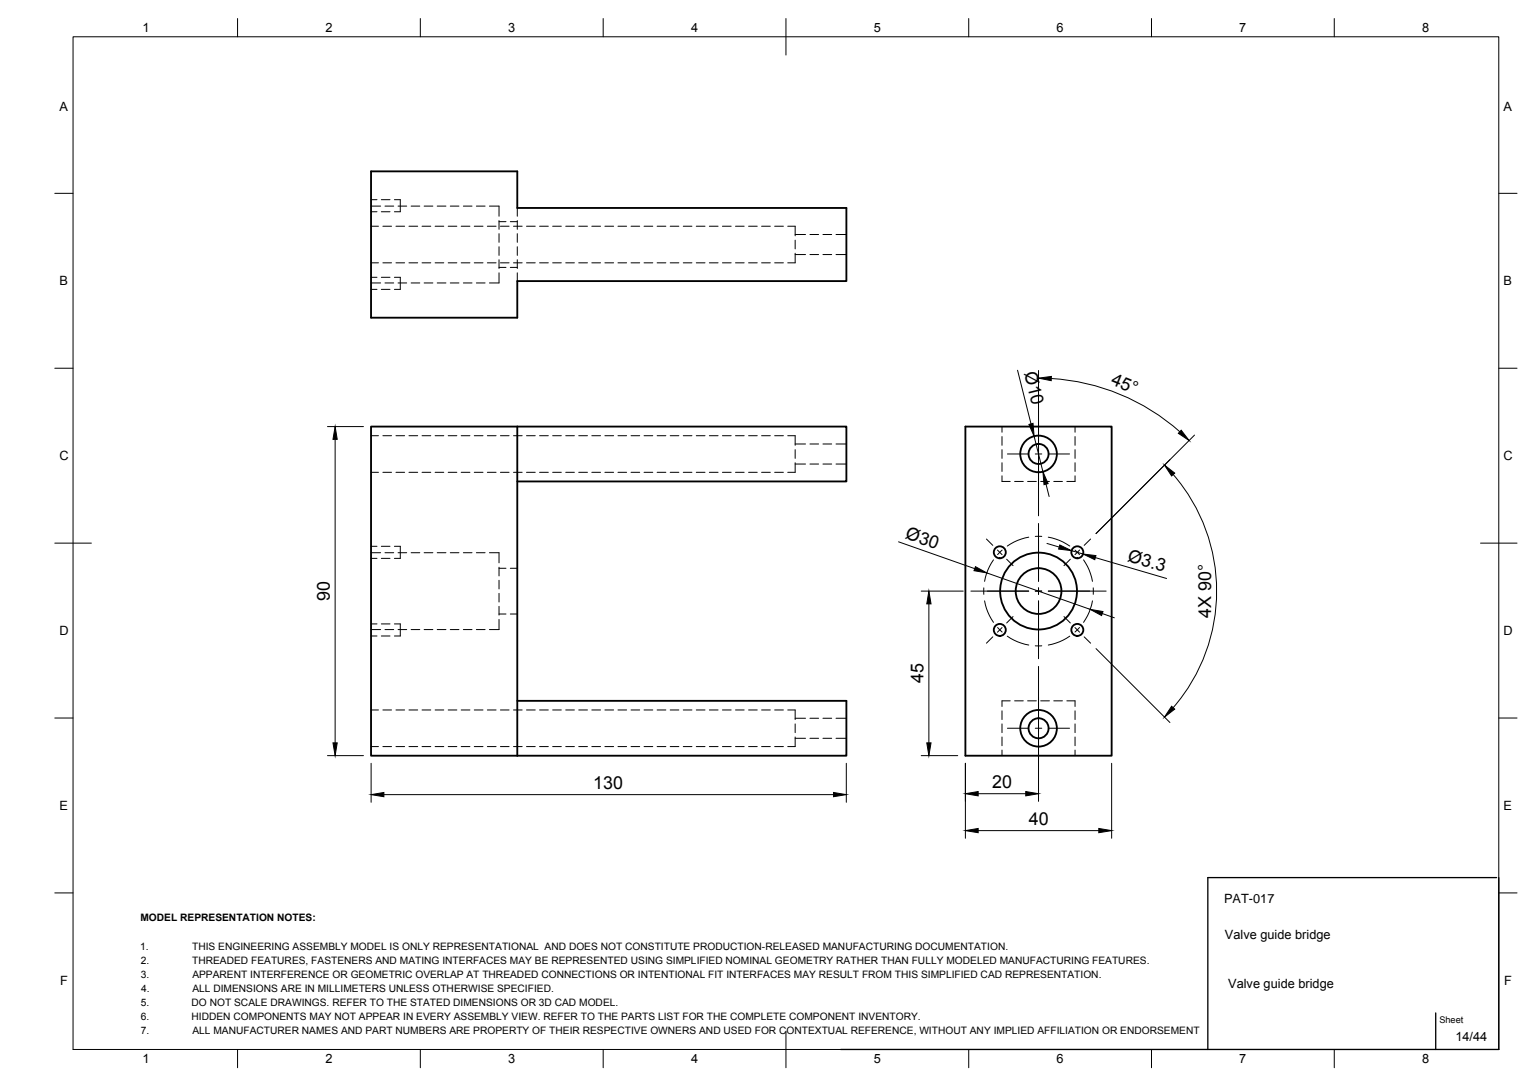
ISO-10303-21;
HEADER;
/* Generated by software containing ST-Developer
 * from STEP Tools, Inc. (www.steptools.com) 
 */

FILE_DESCRIPTION(
/* description */ ('Cam-and-follower valve demonstrator'),
/* implementation_level */ '2;1');

FILE_NAME(
/* name */ 'Valve guide bridge.step',
/* time_stamp */ '2026-10-28T03:25:17-07:00',
/* author */ (''),
/* organization */ (''),
/* preprocessor_version */ 'ST-DEVELOPER v20.2',
/* originating_system */ 'Autodesk Translation Framework v15.17.0.0',
/* authorisation */ '');

FILE_SCHEMA (('AUTOMOTIVE_DESIGN { 1 0 10303 214 3 1 1 }'));
ENDSEC;

DATA;
#10=MECHANICAL_DESIGN_GEOMETRIC_PRESENTATION_REPRESENTATION('',(#421),#12896);
#349=SHAPE_REPRESENTATION_RELATIONSHIP('SRR','None',#13065,#385);
#385=ADVANCED_BREP_SHAPE_REPRESENTATION('',(#464),#12865);
#421=STYLED_ITEM('',(#13323),#464);
#464=MANIFOLD_SOLID_BREP('Body1',#6188);
#580=FACE_BOUND('',#1661,.T.);
#581=FACE_BOUND('',#1665,.T.);
#582=FACE_BOUND('',#1669,.T.);
#583=FACE_BOUND('',#1672,.T.);
#584=FACE_BOUND('',#1678,.T.);
#585=FACE_BOUND('',#1686,.T.);
#586=FACE_BOUND('',#1687,.T.);
#587=FACE_BOUND('',#1688,.T.);
#588=FACE_BOUND('',#1689,.T.);
#589=FACE_BOUND('',#1690,.T.);
#590=FACE_BOUND('',#1691,.T.);
#591=FACE_BOUND('',#1692,.T.);
#592=FACE_BOUND('',#1694,.T.);
#755=CIRCLE('',#6834,0.165);
#756=CIRCLE('',#6835,0.165);
#757=CIRCLE('',#6838,0.165);
#758=CIRCLE('',#6839,0.165);
#759=CIRCLE('',#6842,0.165);
#760=CIRCLE('',#6843,0.165);
#761=CIRCLE('',#6846,0.165);
#762=CIRCLE('',#6847,0.165);
#763=CIRCLE('',#6850,1.05);
#764=CIRCLE('',#6851,1.05);
#765=CIRCLE('',#6853,0.625);
#766=CIRCLE('',#6855,0.625);
#767=CIRCLE('',#6857,0.5);
#768=CIRCLE('',#6858,0.5);
#769=CIRCLE('',#6860,0.275);
#770=CIRCLE('',#6862,0.275);
#771=CIRCLE('',#6864,0.5);
#772=CIRCLE('',#6865,0.5);
#773=CIRCLE('',#6867,0.275);
#774=CIRCLE('',#6869,0.275);
#1021=CYLINDRICAL_SURFACE('',#6833,0.165);
#1022=CYLINDRICAL_SURFACE('',#6837,0.165);
#1023=CYLINDRICAL_SURFACE('',#6841,0.165);
#1024=CYLINDRICAL_SURFACE('',#6845,0.165);
#1025=CYLINDRICAL_SURFACE('',#6849,1.05);
#1026=CYLINDRICAL_SURFACE('',#6854,0.625);
#1027=CYLINDRICAL_SURFACE('',#6856,0.5);
#1028=CYLINDRICAL_SURFACE('',#6861,0.275);
#1029=CYLINDRICAL_SURFACE('',#6863,0.5);
#1030=CYLINDRICAL_SURFACE('',#6868,0.275);
#1198=FACE_OUTER_BOUND('',#1651,.T.);
#1199=FACE_OUTER_BOUND('',#1652,.T.);
#1200=FACE_OUTER_BOUND('',#1653,.T.);
#1201=FACE_OUTER_BOUND('',#1654,.T.);
#1202=FACE_OUTER_BOUND('',#1655,.T.);
#1203=FACE_OUTER_BOUND('',#1656,.T.);
#1204=FACE_OUTER_BOUND('',#1657,.T.);
#1205=FACE_OUTER_BOUND('',#1658,.T.);
#1206=FACE_OUTER_BOUND('',#1659,.T.);
#1207=FACE_OUTER_BOUND('',#1660,.T.);
#1208=FACE_OUTER_BOUND('',#1662,.T.);
#1209=FACE_OUTER_BOUND('',#1663,.T.);
#1210=FACE_OUTER_BOUND('',#1664,.T.);
#1211=FACE_OUTER_BOUND('',#1666,.T.);
#1212=FACE_OUTER_BOUND('',#1667,.T.);
#1213=FACE_OUTER_BOUND('',#1668,.T.);
#1214=FACE_OUTER_BOUND('',#1670,.T.);
#1215=FACE_OUTER_BOUND('',#1671,.T.);
#1216=FACE_OUTER_BOUND('',#1673,.T.);
#1217=FACE_OUTER_BOUND('',#1674,.T.);
#1218=FACE_OUTER_BOUND('',#1675,.T.);
#1219=FACE_OUTER_BOUND('',#1676,.T.);
#1220=FACE_OUTER_BOUND('',#1677,.T.);
#1221=FACE_OUTER_BOUND('',#1679,.T.);
#1222=FACE_OUTER_BOUND('',#1680,.T.);
#1223=FACE_OUTER_BOUND('',#1681,.T.);
#1224=FACE_OUTER_BOUND('',#1682,.T.);
#1225=FACE_OUTER_BOUND('',#1683,.T.);
#1226=FACE_OUTER_BOUND('',#1684,.T.);
#1227=FACE_OUTER_BOUND('',#1685,.T.);
#1228=FACE_OUTER_BOUND('',#1693,.T.);
#1651=EDGE_LOOP('',(#4575,#4576,#4577,#4578));
#1652=EDGE_LOOP('',(#4579));
#1653=EDGE_LOOP('',(#4580,#4581,#4582,#4583));
#1654=EDGE_LOOP('',(#4584));
#1655=EDGE_LOOP('',(#4585,#4586,#4587,#4588));
#1656=EDGE_LOOP('',(#4589));
#1657=EDGE_LOOP('',(#4590,#4591,#4592,#4593));
#1658=EDGE_LOOP('',(#4594));
#1659=EDGE_LOOP('',(#4595,#4596,#4597,#4598));
#1660=EDGE_LOOP('',(#4599));
#1661=EDGE_LOOP('',(#4600));
#1662=EDGE_LOOP('',(#4601,#4602,#4603,#4604));
#1663=EDGE_LOOP('',(#4605,#4606,#4607,#4608));
#1664=EDGE_LOOP('',(#4609));
#1665=EDGE_LOOP('',(#4610));
#1666=EDGE_LOOP('',(#4611,#4612,#4613,#4614));
#1667=EDGE_LOOP('',(#4615,#4616,#4617,#4618));
#1668=EDGE_LOOP('',(#4619));
#1669=EDGE_LOOP('',(#4620));
#1670=EDGE_LOOP('',(#4621,#4622,#4623,#4624));
#1671=EDGE_LOOP('',(#4625,#4626,#4627,#4628,#4629,#4630,#4631,#4632,#4633,
#4634,#4635,#4636));
#1672=EDGE_LOOP('',(#4637));
#1673=EDGE_LOOP('',(#4638,#4639,#4640,#4641));
#1674=EDGE_LOOP('',(#4642,#4643,#4644,#4645));
#1675=EDGE_LOOP('',(#4646,#4647,#4648,#4649));
#1676=EDGE_LOOP('',(#4650,#4651,#4652,#4653));
#1677=EDGE_LOOP('',(#4654,#4655,#4656,#4657));
#1678=EDGE_LOOP('',(#4658));
#1679=EDGE_LOOP('',(#4659,#4660,#4661,#4662,#4663,#4664,#4665,#4666));
#1680=EDGE_LOOP('',(#4667,#4668,#4669,#4670));
#1681=EDGE_LOOP('',(#4671,#4672,#4673,#4674));
#1682=EDGE_LOOP('',(#4675,#4676,#4677,#4678));
#1683=EDGE_LOOP('',(#4679,#4680,#4681,#4682));
#1684=EDGE_LOOP('',(#4683,#4684,#4685,#4686,#4687,#4688,#4689,#4690));
#1685=EDGE_LOOP('',(#4691,#4692,#4693,#4694));
#1686=EDGE_LOOP('',(#4695));
#1687=EDGE_LOOP('',(#4696));
#1688=EDGE_LOOP('',(#4697));
#1689=EDGE_LOOP('',(#4698));
#1690=EDGE_LOOP('',(#4699));
#1691=EDGE_LOOP('',(#4700));
#1692=EDGE_LOOP('',(#4701));
#1693=EDGE_LOOP('',(#4702,#4703,#4704,#4705));
#1694=EDGE_LOOP('',(#4706));
#2139=LINE('',#9939,#2561);
#2140=LINE('',#9946,#2562);
#2141=LINE('',#9953,#2563);
#2142=LINE('',#9960,#2564);
#2143=LINE('',#9967,#2565);
#2144=LINE('',#9975,#2566);
#2145=LINE('',#9980,#2567);
#2146=LINE('',#9988,#2568);
#2147=LINE('',#9993,#2569);
#2148=LINE('',#10001,#2570);
#2149=LINE('',#10005,#2571);
#2150=LINE('',#10007,#2572);
#2151=LINE('',#10009,#2573);
#2152=LINE('',#10011,#2574);
#2153=LINE('',#10013,#2575);
#2154=LINE('',#10015,#2576);
#2155=LINE('',#10017,#2577);
#2156=LINE('',#10019,#2578);
#2157=LINE('',#10021,#2579);
#2158=LINE('',#10023,#2580);
#2159=LINE('',#10025,#2581);
#2160=LINE('',#10026,#2582);
#2161=LINE('',#10030,#2583);
#2162=LINE('',#10031,#2584);
#2163=LINE('',#10032,#2585);
#2164=LINE('',#10036,#2586);
#2165=LINE('',#10037,#2587);
#2166=LINE('',#10038,#2588);
#2167=LINE('',#10041,#2589);
#2168=LINE('',#10043,#2590);
#2169=LINE('',#10044,#2591);
#2170=LINE('',#10047,#2592);
#2171=LINE('',#10048,#2593);
#2172=LINE('',#10051,#2594);
#2173=LINE('',#10052,#2595);
#2174=LINE('',#10054,#2596);
#2175=LINE('',#10055,#2597);
#2176=LINE('',#10059,#2598);
#2177=LINE('',#10061,#2599);
#2178=LINE('',#10062,#2600);
#2179=LINE('',#10065,#2601);
#2180=LINE('',#10066,#2602);
#2181=LINE('',#10069,#2603);
#2182=LINE('',#10070,#2604);
#2183=LINE('',#10072,#2605);
#2184=LINE('',#10073,#2606);
#2561=VECTOR('',#7984,0.165);
#2562=VECTOR('',#7993,0.165);
#2563=VECTOR('',#8002,0.165);
#2564=VECTOR('',#8011,0.165);
#2565=VECTOR('',#8020,1.05);
#2566=VECTOR('',#8031,0.625);
#2567=VECTOR('',#8036,0.5);
#2568=VECTOR('',#8047,0.275);
#2569=VECTOR('',#8052,0.5);
#2570=VECTOR('',#8063,0.275);
#2571=VECTOR('',#8066,1.);
#2572=VECTOR('',#8067,1.);
#2573=VECTOR('',#8068,1.);
#2574=VECTOR('',#8069,1.);
#2575=VECTOR('',#8070,1.);
#2576=VECTOR('',#8071,1.);
#2577=VECTOR('',#8072,1.);
#2578=VECTOR('',#8073,1.);
#2579=VECTOR('',#8074,1.);
#2580=VECTOR('',#8075,1.);
#2581=VECTOR('',#8076,1.);
#2582=VECTOR('',#8077,1.);
#2583=VECTOR('',#8080,1.);
#2584=VECTOR('',#8081,1.);
#2585=VECTOR('',#8082,1.);
#2586=VECTOR('',#8085,1.);
#2587=VECTOR('',#8086,1.);
#2588=VECTOR('',#8087,1.);
#2589=VECTOR('',#8090,1.);
#2590=VECTOR('',#8091,1.);
#2591=VECTOR('',#8092,1.);
#2592=VECTOR('',#8095,1.);
#2593=VECTOR('',#8096,1.);
#2594=VECTOR('',#8099,1.);
#2595=VECTOR('',#8100,1.);
#2596=VECTOR('',#8103,1.);
#2597=VECTOR('',#8104,1.);
#2598=VECTOR('',#8109,1.);
#2599=VECTOR('',#8110,1.);
#2600=VECTOR('',#8111,1.);
#2601=VECTOR('',#8114,1.);
#2602=VECTOR('',#8115,1.);
#2603=VECTOR('',#8118,1.);
#2604=VECTOR('',#8119,1.);
#2605=VECTOR('',#8122,1.);
#2606=VECTOR('',#8123,1.);
#2999=VERTEX_POINT('',#9936);
#3000=VERTEX_POINT('',#9938);
#3001=VERTEX_POINT('',#9943);
#3002=VERTEX_POINT('',#9945);
#3003=VERTEX_POINT('',#9950);
#3004=VERTEX_POINT('',#9952);
#3005=VERTEX_POINT('',#9957);
#3006=VERTEX_POINT('',#9959);
#3007=VERTEX_POINT('',#9964);
#3008=VERTEX_POINT('',#9966);
#3009=VERTEX_POINT('',#9970);
#3010=VERTEX_POINT('',#9973);
#3011=VERTEX_POINT('',#9977);
#3012=VERTEX_POINT('',#9979);
#3013=VERTEX_POINT('',#9983);
#3014=VERTEX_POINT('',#9986);
#3015=VERTEX_POINT('',#9990);
#3016=VERTEX_POINT('',#9992);
#3017=VERTEX_POINT('',#9996);
#3018=VERTEX_POINT('',#9999);
#3019=VERTEX_POINT('',#10003);
#3020=VERTEX_POINT('',#10004);
#3021=VERTEX_POINT('',#10006);
#3022=VERTEX_POINT('',#10008);
#3023=VERTEX_POINT('',#10010);
#3024=VERTEX_POINT('',#10012);
#3025=VERTEX_POINT('',#10014);
#3026=VERTEX_POINT('',#10016);
#3027=VERTEX_POINT('',#10018);
#3028=VERTEX_POINT('',#10020);
#3029=VERTEX_POINT('',#10022);
#3030=VERTEX_POINT('',#10024);
#3031=VERTEX_POINT('',#10028);
#3032=VERTEX_POINT('',#10029);
#3033=VERTEX_POINT('',#10034);
#3034=VERTEX_POINT('',#10035);
#3035=VERTEX_POINT('',#10040);
#3036=VERTEX_POINT('',#10042);
#3037=VERTEX_POINT('',#10046);
#3038=VERTEX_POINT('',#10050);
#3039=VERTEX_POINT('',#10058);
#3040=VERTEX_POINT('',#10060);
#3041=VERTEX_POINT('',#10064);
#3042=VERTEX_POINT('',#10068);
#3584=EDGE_CURVE('',#2999,#2999,#755,.T.);
#3585=EDGE_CURVE('',#2999,#3000,#2139,.T.);
#3586=EDGE_CURVE('',#3000,#3000,#756,.T.);
#3587=EDGE_CURVE('',#3001,#3001,#757,.T.);
#3588=EDGE_CURVE('',#3001,#3002,#2140,.T.);
#3589=EDGE_CURVE('',#3002,#3002,#758,.T.);
#3590=EDGE_CURVE('',#3003,#3003,#759,.T.);
#3591=EDGE_CURVE('',#3003,#3004,#2141,.T.);
#3592=EDGE_CURVE('',#3004,#3004,#760,.T.);
#3593=EDGE_CURVE('',#3005,#3005,#761,.T.);
#3594=EDGE_CURVE('',#3005,#3006,#2142,.T.);
#3595=EDGE_CURVE('',#3006,#3006,#762,.T.);
#3596=EDGE_CURVE('',#3007,#3007,#763,.T.);
#3597=EDGE_CURVE('',#3007,#3008,#2143,.T.);
#3598=EDGE_CURVE('',#3008,#3008,#764,.T.);
#3599=EDGE_CURVE('',#3009,#3009,#765,.T.);
#3600=EDGE_CURVE('',#3010,#3010,#766,.T.);
#3601=EDGE_CURVE('',#3010,#3009,#2144,.T.);
#3602=EDGE_CURVE('',#3011,#3011,#767,.T.);
#3603=EDGE_CURVE('',#3011,#3012,#2145,.T.);
#3604=EDGE_CURVE('',#3012,#3012,#768,.T.);
#3605=EDGE_CURVE('',#3013,#3013,#769,.T.);
#3606=EDGE_CURVE('',#3014,#3014,#770,.T.);
#3607=EDGE_CURVE('',#3014,#3013,#2146,.T.);
#3608=EDGE_CURVE('',#3015,#3015,#771,.T.);
#3609=EDGE_CURVE('',#3015,#3016,#2147,.T.);
#3610=EDGE_CURVE('',#3016,#3016,#772,.T.);
#3611=EDGE_CURVE('',#3017,#3017,#773,.T.);
#3612=EDGE_CURVE('',#3018,#3018,#774,.T.);
#3613=EDGE_CURVE('',#3018,#3017,#2148,.T.);
#3614=EDGE_CURVE('',#3019,#3020,#2149,.T.);
#3615=EDGE_CURVE('',#3019,#3021,#2150,.T.);
#3616=EDGE_CURVE('',#3022,#3021,#2151,.T.);
#3617=EDGE_CURVE('',#3023,#3022,#2152,.T.);
#3618=EDGE_CURVE('',#3024,#3023,#2153,.T.);
#3619=EDGE_CURVE('',#3025,#3024,#2154,.T.);
#3620=EDGE_CURVE('',#3026,#3025,#2155,.T.);
#3621=EDGE_CURVE('',#3027,#3026,#2156,.T.);
#3622=EDGE_CURVE('',#3028,#3027,#2157,.T.);
#3623=EDGE_CURVE('',#3028,#3029,#2158,.T.);
#3624=EDGE_CURVE('',#3030,#3029,#2159,.T.);
#3625=EDGE_CURVE('',#3020,#3030,#2160,.T.);
#3626=EDGE_CURVE('',#3031,#3032,#2161,.T.);
#3627=EDGE_CURVE('',#3032,#3022,#2162,.T.);
#3628=EDGE_CURVE('',#3021,#3031,#2163,.T.);
#3629=EDGE_CURVE('',#3033,#3034,#2164,.T.);
#3630=EDGE_CURVE('',#3034,#3028,#2165,.T.);
#3631=EDGE_CURVE('',#3027,#3033,#2166,.T.);
#3632=EDGE_CURVE('',#3035,#3024,#2167,.T.);
#3633=EDGE_CURVE('',#3036,#3035,#2168,.T.);
#3634=EDGE_CURVE('',#3025,#3036,#2169,.T.);
#3635=EDGE_CURVE('',#3023,#3037,#2170,.T.);
#3636=EDGE_CURVE('',#3037,#3035,#2171,.T.);
#3637=EDGE_CURVE('',#3036,#3038,#2172,.T.);
#3638=EDGE_CURVE('',#3038,#3037,#2173,.T.);
#3639=EDGE_CURVE('',#3038,#3026,#2174,.T.);
#3640=EDGE_CURVE('',#3033,#3032,#2175,.T.);
#3641=EDGE_CURVE('',#3039,#3030,#2176,.T.);
#3642=EDGE_CURVE('',#3039,#3040,#2177,.T.);
#3643=EDGE_CURVE('',#3040,#3020,#2178,.T.);
#3644=EDGE_CURVE('',#3041,#3029,#2179,.T.);
#3645=EDGE_CURVE('',#3041,#3039,#2180,.T.);
#3646=EDGE_CURVE('',#3040,#3042,#2181,.T.);
#3647=EDGE_CURVE('',#3042,#3019,#2182,.T.);
#3648=EDGE_CURVE('',#3042,#3041,#2183,.T.);
#3649=EDGE_CURVE('',#3034,#3031,#2184,.T.);
#4575=ORIENTED_EDGE('',*,*,#3584,.F.);
#4576=ORIENTED_EDGE('',*,*,#3585,.T.);
#4577=ORIENTED_EDGE('',*,*,#3586,.F.);
#4578=ORIENTED_EDGE('',*,*,#3585,.F.);
#4579=ORIENTED_EDGE('',*,*,#3584,.T.);
#4580=ORIENTED_EDGE('',*,*,#3587,.F.);
#4581=ORIENTED_EDGE('',*,*,#3588,.T.);
#4582=ORIENTED_EDGE('',*,*,#3589,.F.);
#4583=ORIENTED_EDGE('',*,*,#3588,.F.);
#4584=ORIENTED_EDGE('',*,*,#3587,.T.);
#4585=ORIENTED_EDGE('',*,*,#3590,.F.);
#4586=ORIENTED_EDGE('',*,*,#3591,.T.);
#4587=ORIENTED_EDGE('',*,*,#3592,.F.);
#4588=ORIENTED_EDGE('',*,*,#3591,.F.);
#4589=ORIENTED_EDGE('',*,*,#3590,.T.);
#4590=ORIENTED_EDGE('',*,*,#3593,.F.);
#4591=ORIENTED_EDGE('',*,*,#3594,.T.);
#4592=ORIENTED_EDGE('',*,*,#3595,.F.);
#4593=ORIENTED_EDGE('',*,*,#3594,.F.);
#4594=ORIENTED_EDGE('',*,*,#3593,.T.);
#4595=ORIENTED_EDGE('',*,*,#3596,.F.);
#4596=ORIENTED_EDGE('',*,*,#3597,.T.);
#4597=ORIENTED_EDGE('',*,*,#3598,.F.);
#4598=ORIENTED_EDGE('',*,*,#3597,.F.);
#4599=ORIENTED_EDGE('',*,*,#3596,.T.);
#4600=ORIENTED_EDGE('',*,*,#3599,.F.);
#4601=ORIENTED_EDGE('',*,*,#3600,.F.);
#4602=ORIENTED_EDGE('',*,*,#3601,.T.);
#4603=ORIENTED_EDGE('',*,*,#3599,.T.);
#4604=ORIENTED_EDGE('',*,*,#3601,.F.);
#4605=ORIENTED_EDGE('',*,*,#3602,.F.);
#4606=ORIENTED_EDGE('',*,*,#3603,.T.);
#4607=ORIENTED_EDGE('',*,*,#3604,.F.);
#4608=ORIENTED_EDGE('',*,*,#3603,.F.);
#4609=ORIENTED_EDGE('',*,*,#3602,.T.);
#4610=ORIENTED_EDGE('',*,*,#3605,.F.);
#4611=ORIENTED_EDGE('',*,*,#3606,.F.);
#4612=ORIENTED_EDGE('',*,*,#3607,.T.);
#4613=ORIENTED_EDGE('',*,*,#3605,.T.);
#4614=ORIENTED_EDGE('',*,*,#3607,.F.);
#4615=ORIENTED_EDGE('',*,*,#3608,.F.);
#4616=ORIENTED_EDGE('',*,*,#3609,.T.);
#4617=ORIENTED_EDGE('',*,*,#3610,.F.);
#4618=ORIENTED_EDGE('',*,*,#3609,.F.);
#4619=ORIENTED_EDGE('',*,*,#3608,.T.);
#4620=ORIENTED_EDGE('',*,*,#3611,.F.);
#4621=ORIENTED_EDGE('',*,*,#3612,.F.);
#4622=ORIENTED_EDGE('',*,*,#3613,.T.);
#4623=ORIENTED_EDGE('',*,*,#3611,.T.);
#4624=ORIENTED_EDGE('',*,*,#3613,.F.);
#4625=ORIENTED_EDGE('',*,*,#3614,.F.);
#4626=ORIENTED_EDGE('',*,*,#3615,.T.);
#4627=ORIENTED_EDGE('',*,*,#3616,.F.);
#4628=ORIENTED_EDGE('',*,*,#3617,.F.);
#4629=ORIENTED_EDGE('',*,*,#3618,.F.);
#4630=ORIENTED_EDGE('',*,*,#3619,.F.);
#4631=ORIENTED_EDGE('',*,*,#3620,.F.);
#4632=ORIENTED_EDGE('',*,*,#3621,.F.);
#4633=ORIENTED_EDGE('',*,*,#3622,.F.);
#4634=ORIENTED_EDGE('',*,*,#3623,.T.);
#4635=ORIENTED_EDGE('',*,*,#3624,.F.);
#4636=ORIENTED_EDGE('',*,*,#3625,.F.);
#4637=ORIENTED_EDGE('',*,*,#3600,.T.);
#4638=ORIENTED_EDGE('',*,*,#3626,.T.);
#4639=ORIENTED_EDGE('',*,*,#3627,.T.);
#4640=ORIENTED_EDGE('',*,*,#3616,.T.);
#4641=ORIENTED_EDGE('',*,*,#3628,.T.);
#4642=ORIENTED_EDGE('',*,*,#3629,.T.);
#4643=ORIENTED_EDGE('',*,*,#3630,.T.);
#4644=ORIENTED_EDGE('',*,*,#3622,.T.);
#4645=ORIENTED_EDGE('',*,*,#3631,.T.);
#4646=ORIENTED_EDGE('',*,*,#3619,.T.);
#4647=ORIENTED_EDGE('',*,*,#3632,.F.);
#4648=ORIENTED_EDGE('',*,*,#3633,.F.);
#4649=ORIENTED_EDGE('',*,*,#3634,.F.);
#4650=ORIENTED_EDGE('',*,*,#3618,.T.);
#4651=ORIENTED_EDGE('',*,*,#3635,.T.);
#4652=ORIENTED_EDGE('',*,*,#3636,.T.);
#4653=ORIENTED_EDGE('',*,*,#3632,.T.);
#4654=ORIENTED_EDGE('',*,*,#3637,.F.);
#4655=ORIENTED_EDGE('',*,*,#3633,.T.);
#4656=ORIENTED_EDGE('',*,*,#3636,.F.);
#4657=ORIENTED_EDGE('',*,*,#3638,.F.);
#4658=ORIENTED_EDGE('',*,*,#3606,.T.);
#4659=ORIENTED_EDGE('',*,*,#3639,.F.);
#4660=ORIENTED_EDGE('',*,*,#3638,.T.);
#4661=ORIENTED_EDGE('',*,*,#3635,.F.);
#4662=ORIENTED_EDGE('',*,*,#3617,.T.);
#4663=ORIENTED_EDGE('',*,*,#3627,.F.);
#4664=ORIENTED_EDGE('',*,*,#3640,.F.);
#4665=ORIENTED_EDGE('',*,*,#3631,.F.);
#4666=ORIENTED_EDGE('',*,*,#3621,.T.);
#4667=ORIENTED_EDGE('',*,*,#3620,.T.);
#4668=ORIENTED_EDGE('',*,*,#3634,.T.);
#4669=ORIENTED_EDGE('',*,*,#3637,.T.);
#4670=ORIENTED_EDGE('',*,*,#3639,.T.);
#4671=ORIENTED_EDGE('',*,*,#3625,.T.);
#4672=ORIENTED_EDGE('',*,*,#3641,.F.);
#4673=ORIENTED_EDGE('',*,*,#3642,.T.);
#4674=ORIENTED_EDGE('',*,*,#3643,.T.);
#4675=ORIENTED_EDGE('',*,*,#3624,.T.);
#4676=ORIENTED_EDGE('',*,*,#3644,.F.);
#4677=ORIENTED_EDGE('',*,*,#3645,.T.);
#4678=ORIENTED_EDGE('',*,*,#3641,.T.);
#4679=ORIENTED_EDGE('',*,*,#3614,.T.);
#4680=ORIENTED_EDGE('',*,*,#3643,.F.);
#4681=ORIENTED_EDGE('',*,*,#3646,.T.);
#4682=ORIENTED_EDGE('',*,*,#3647,.T.);
#4683=ORIENTED_EDGE('',*,*,#3647,.F.);
#4684=ORIENTED_EDGE('',*,*,#3648,.T.);
#4685=ORIENTED_EDGE('',*,*,#3644,.T.);
#4686=ORIENTED_EDGE('',*,*,#3623,.F.);
#4687=ORIENTED_EDGE('',*,*,#3630,.F.);
#4688=ORIENTED_EDGE('',*,*,#3649,.T.);
#4689=ORIENTED_EDGE('',*,*,#3628,.F.);
#4690=ORIENTED_EDGE('',*,*,#3615,.F.);
#4691=ORIENTED_EDGE('',*,*,#3649,.F.);
#4692=ORIENTED_EDGE('',*,*,#3629,.F.);
#4693=ORIENTED_EDGE('',*,*,#3640,.T.);
#4694=ORIENTED_EDGE('',*,*,#3626,.F.);
#4695=ORIENTED_EDGE('',*,*,#3610,.T.);
#4696=ORIENTED_EDGE('',*,*,#3604,.T.);
#4697=ORIENTED_EDGE('',*,*,#3598,.T.);
#4698=ORIENTED_EDGE('',*,*,#3595,.T.);
#4699=ORIENTED_EDGE('',*,*,#3592,.T.);
#4700=ORIENTED_EDGE('',*,*,#3589,.T.);
#4701=ORIENTED_EDGE('',*,*,#3586,.T.);
#4702=ORIENTED_EDGE('',*,*,#3648,.F.);
#4703=ORIENTED_EDGE('',*,*,#3646,.F.);
#4704=ORIENTED_EDGE('',*,*,#3642,.F.);
#4705=ORIENTED_EDGE('',*,*,#3645,.F.);
#4706=ORIENTED_EDGE('',*,*,#3612,.T.);
#5652=PLANE('',#6836);
#5653=PLANE('',#6840);
#5654=PLANE('',#6844);
#5655=PLANE('',#6848);
#5656=PLANE('',#6852);
#5657=PLANE('',#6859);
#5658=PLANE('',#6866);
#5659=PLANE('',#6870);
#5660=PLANE('',#6871);
#5661=PLANE('',#6872);
#5662=PLANE('',#6873);
#5663=PLANE('',#6874);
#5664=PLANE('',#6875);
#5665=PLANE('',#6876);
#5666=PLANE('',#6877);
#5667=PLANE('',#6878);
#5668=PLANE('',#6879);
#5669=PLANE('',#6880);
#5670=PLANE('',#6881);
#5671=PLANE('',#6882);
#5672=PLANE('',#6883);
#5914=ADVANCED_FACE('',(#1198),#1021,.F.);
#5915=ADVANCED_FACE('',(#1199),#5652,.T.);
#5916=ADVANCED_FACE('',(#1200),#1022,.F.);
#5917=ADVANCED_FACE('',(#1201),#5653,.T.);
#5918=ADVANCED_FACE('',(#1202),#1023,.F.);
#5919=ADVANCED_FACE('',(#1203),#5654,.T.);
#5920=ADVANCED_FACE('',(#1204),#1024,.F.);
#5921=ADVANCED_FACE('',(#1205),#5655,.T.);
#5922=ADVANCED_FACE('',(#1206),#1025,.F.);
#5923=ADVANCED_FACE('',(#1207,#580),#5656,.T.);
#5924=ADVANCED_FACE('',(#1208),#1026,.F.);
#5925=ADVANCED_FACE('',(#1209),#1027,.F.);
#5926=ADVANCED_FACE('',(#1210,#581),#5657,.T.);
#5927=ADVANCED_FACE('',(#1211),#1028,.F.);
#5928=ADVANCED_FACE('',(#1212),#1029,.F.);
#5929=ADVANCED_FACE('',(#1213,#582),#5658,.T.);
#5930=ADVANCED_FACE('',(#1214),#1030,.F.);
#5931=ADVANCED_FACE('',(#1215,#583),#5659,.T.);
#5932=ADVANCED_FACE('',(#1216),#5660,.T.);
#5933=ADVANCED_FACE('',(#1217),#5661,.F.);
#5934=ADVANCED_FACE('',(#1218),#5662,.T.);
#5935=ADVANCED_FACE('',(#1219),#5663,.T.);
#5936=ADVANCED_FACE('',(#1220,#584),#5664,.T.);
#5937=ADVANCED_FACE('',(#1221),#5665,.T.);
#5938=ADVANCED_FACE('',(#1222),#5666,.F.);
#5939=ADVANCED_FACE('',(#1223),#5667,.T.);
#5940=ADVANCED_FACE('',(#1224),#5668,.T.);
#5941=ADVANCED_FACE('',(#1225),#5669,.T.);
#5942=ADVANCED_FACE('',(#1226),#5670,.T.);
#5943=ADVANCED_FACE('',(#1227,#585,#586,#587,#588,#589,#590,#591),#5671,
 .T.);
#5944=ADVANCED_FACE('',(#1228,#592),#5672,.F.);
#6188=CLOSED_SHELL('',(#5914,#5915,#5916,#5917,#5918,#5919,#5920,#5921,
#5922,#5923,#5924,#5925,#5926,#5927,#5928,#5929,#5930,#5931,#5932,#5933,
#5934,#5935,#5936,#5937,#5938,#5939,#5940,#5941,#5942,#5943,#5944));
#6832=AXIS2_PLACEMENT_3D('',#9934,#7978,#7979);
#6833=AXIS2_PLACEMENT_3D('',#9935,#7980,#7981);
#6834=AXIS2_PLACEMENT_3D('',#9937,#7982,#7983);
#6835=AXIS2_PLACEMENT_3D('',#9940,#7985,#7986);
#6836=AXIS2_PLACEMENT_3D('',#9941,#7987,#7988);
#6837=AXIS2_PLACEMENT_3D('',#9942,#7989,#7990);
#6838=AXIS2_PLACEMENT_3D('',#9944,#7991,#7992);
#6839=AXIS2_PLACEMENT_3D('',#9947,#7994,#7995);
#6840=AXIS2_PLACEMENT_3D('',#9948,#7996,#7997);
#6841=AXIS2_PLACEMENT_3D('',#9949,#7998,#7999);
#6842=AXIS2_PLACEMENT_3D('',#9951,#8000,#8001);
#6843=AXIS2_PLACEMENT_3D('',#9954,#8003,#8004);
#6844=AXIS2_PLACEMENT_3D('',#9955,#8005,#8006);
#6845=AXIS2_PLACEMENT_3D('',#9956,#8007,#8008);
#6846=AXIS2_PLACEMENT_3D('',#9958,#8009,#8010);
#6847=AXIS2_PLACEMENT_3D('',#9961,#8012,#8013);
#6848=AXIS2_PLACEMENT_3D('',#9962,#8014,#8015);
#6849=AXIS2_PLACEMENT_3D('',#9963,#8016,#8017);
#6850=AXIS2_PLACEMENT_3D('',#9965,#8018,#8019);
#6851=AXIS2_PLACEMENT_3D('',#9968,#8021,#8022);
#6852=AXIS2_PLACEMENT_3D('',#9969,#8023,#8024);
#6853=AXIS2_PLACEMENT_3D('',#9971,#8025,#8026);
#6854=AXIS2_PLACEMENT_3D('',#9972,#8027,#8028);
#6855=AXIS2_PLACEMENT_3D('',#9974,#8029,#8030);
#6856=AXIS2_PLACEMENT_3D('',#9976,#8032,#8033);
#6857=AXIS2_PLACEMENT_3D('',#9978,#8034,#8035);
#6858=AXIS2_PLACEMENT_3D('',#9981,#8037,#8038);
#6859=AXIS2_PLACEMENT_3D('',#9982,#8039,#8040);
#6860=AXIS2_PLACEMENT_3D('',#9984,#8041,#8042);
#6861=AXIS2_PLACEMENT_3D('',#9985,#8043,#8044);
#6862=AXIS2_PLACEMENT_3D('',#9987,#8045,#8046);
#6863=AXIS2_PLACEMENT_3D('',#9989,#8048,#8049);
#6864=AXIS2_PLACEMENT_3D('',#9991,#8050,#8051);
#6865=AXIS2_PLACEMENT_3D('',#9994,#8053,#8054);
#6866=AXIS2_PLACEMENT_3D('',#9995,#8055,#8056);
#6867=AXIS2_PLACEMENT_3D('',#9997,#8057,#8058);
#6868=AXIS2_PLACEMENT_3D('',#9998,#8059,#8060);
#6869=AXIS2_PLACEMENT_3D('',#10000,#8061,#8062);
#6870=AXIS2_PLACEMENT_3D('',#10002,#8064,#8065);
#6871=AXIS2_PLACEMENT_3D('',#10027,#8078,#8079);
#6872=AXIS2_PLACEMENT_3D('',#10033,#8083,#8084);
#6873=AXIS2_PLACEMENT_3D('',#10039,#8088,#8089);
#6874=AXIS2_PLACEMENT_3D('',#10045,#8093,#8094);
#6875=AXIS2_PLACEMENT_3D('',#10049,#8097,#8098);
#6876=AXIS2_PLACEMENT_3D('',#10053,#8101,#8102);
#6877=AXIS2_PLACEMENT_3D('',#10056,#8105,#8106);
#6878=AXIS2_PLACEMENT_3D('',#10057,#8107,#8108);
#6879=AXIS2_PLACEMENT_3D('',#10063,#8112,#8113);
#6880=AXIS2_PLACEMENT_3D('',#10067,#8116,#8117);
#6881=AXIS2_PLACEMENT_3D('',#10071,#8120,#8121);
#6882=AXIS2_PLACEMENT_3D('',#10074,#8124,#8125);
#6883=AXIS2_PLACEMENT_3D('',#10075,#8126,#8127);
#7978=DIRECTION('axis',(0.,0.,1.));
#7979=DIRECTION('refdir',(1.,0.,0.));
#7980=DIRECTION('center_axis',(0.,0.,1.));
#7981=DIRECTION('ref_axis',(1.,0.,0.));
#7982=DIRECTION('center_axis',(0.,0.,1.));
#7983=DIRECTION('ref_axis',(1.,0.,0.));
#7984=DIRECTION('',(0.,0.,1.));
#7985=DIRECTION('center_axis',(0.,0.,-1.));
#7986=DIRECTION('ref_axis',(1.,0.,0.));
#7987=DIRECTION('center_axis',(0.,0.,1.));
#7988=DIRECTION('ref_axis',(1.,0.,0.));
#7989=DIRECTION('center_axis',(0.,0.,1.));
#7990=DIRECTION('ref_axis',(1.,0.,0.));
#7991=DIRECTION('center_axis',(0.,0.,1.));
#7992=DIRECTION('ref_axis',(1.,0.,0.));
#7993=DIRECTION('',(0.,0.,1.));
#7994=DIRECTION('center_axis',(0.,0.,-1.));
#7995=DIRECTION('ref_axis',(1.,0.,0.));
#7996=DIRECTION('center_axis',(0.,0.,1.));
#7997=DIRECTION('ref_axis',(1.,0.,0.));
#7998=DIRECTION('center_axis',(0.,0.,1.));
#7999=DIRECTION('ref_axis',(1.,0.,0.));
#8000=DIRECTION('center_axis',(0.,0.,1.));
#8001=DIRECTION('ref_axis',(1.,0.,0.));
#8002=DIRECTION('',(0.,0.,1.));
#8003=DIRECTION('center_axis',(0.,0.,-1.));
#8004=DIRECTION('ref_axis',(1.,0.,0.));
#8005=DIRECTION('center_axis',(0.,0.,1.));
#8006=DIRECTION('ref_axis',(1.,0.,0.));
#8007=DIRECTION('center_axis',(0.,0.,1.));
#8008=DIRECTION('ref_axis',(1.,0.,0.));
#8009=DIRECTION('center_axis',(0.,0.,1.));
#8010=DIRECTION('ref_axis',(1.,0.,0.));
#8011=DIRECTION('',(0.,0.,1.));
#8012=DIRECTION('center_axis',(0.,0.,-1.));
#8013=DIRECTION('ref_axis',(1.,0.,0.));
#8014=DIRECTION('center_axis',(0.,0.,1.));
#8015=DIRECTION('ref_axis',(1.,0.,0.));
#8016=DIRECTION('center_axis',(0.,0.,1.));
#8017=DIRECTION('ref_axis',(1.,0.,0.));
#8018=DIRECTION('center_axis',(0.,0.,1.));
#8019=DIRECTION('ref_axis',(1.,0.,0.));
#8020=DIRECTION('',(0.,0.,1.));
#8021=DIRECTION('center_axis',(0.,0.,-1.));
#8022=DIRECTION('ref_axis',(1.,0.,0.));
#8023=DIRECTION('center_axis',(0.,0.,1.));
#8024=DIRECTION('ref_axis',(1.,0.,0.));
#8025=DIRECTION('center_axis',(0.,0.,1.));
#8026=DIRECTION('ref_axis',(1.,0.,0.));
#8027=DIRECTION('center_axis',(0.,0.,1.));
#8028=DIRECTION('ref_axis',(1.,0.,0.));
#8029=DIRECTION('center_axis',(0.,0.,1.));
#8030=DIRECTION('ref_axis',(1.,0.,0.));
#8031=DIRECTION('',(0.,0.,1.));
#8032=DIRECTION('center_axis',(0.,0.,1.));
#8033=DIRECTION('ref_axis',(1.,0.,0.));
#8034=DIRECTION('center_axis',(0.,0.,1.));
#8035=DIRECTION('ref_axis',(1.,0.,0.));
#8036=DIRECTION('',(0.,0.,1.));
#8037=DIRECTION('center_axis',(0.,0.,-1.));
#8038=DIRECTION('ref_axis',(1.,0.,0.));
#8039=DIRECTION('center_axis',(0.,0.,1.));
#8040=DIRECTION('ref_axis',(1.,0.,0.));
#8041=DIRECTION('center_axis',(0.,0.,1.));
#8042=DIRECTION('ref_axis',(1.,0.,0.));
#8043=DIRECTION('center_axis',(0.,0.,1.));
#8044=DIRECTION('ref_axis',(1.,0.,0.));
#8045=DIRECTION('center_axis',(0.,0.,1.));
#8046=DIRECTION('ref_axis',(1.,0.,0.));
#8047=DIRECTION('',(0.,0.,1.));
#8048=DIRECTION('center_axis',(0.,0.,1.));
#8049=DIRECTION('ref_axis',(1.,0.,0.));
#8050=DIRECTION('center_axis',(0.,0.,1.));
#8051=DIRECTION('ref_axis',(1.,0.,0.));
#8052=DIRECTION('',(0.,0.,1.));
#8053=DIRECTION('center_axis',(0.,0.,-1.));
#8054=DIRECTION('ref_axis',(1.,0.,0.));
#8055=DIRECTION('center_axis',(0.,0.,1.));
#8056=DIRECTION('ref_axis',(1.,0.,0.));
#8057=DIRECTION('center_axis',(0.,0.,1.));
#8058=DIRECTION('ref_axis',(1.,0.,0.));
#8059=DIRECTION('center_axis',(0.,0.,1.));
#8060=DIRECTION('ref_axis',(1.,0.,0.));
#8061=DIRECTION('center_axis',(0.,0.,1.));
#8062=DIRECTION('ref_axis',(1.,0.,0.));
#8063=DIRECTION('',(0.,0.,1.));
#8064=DIRECTION('center_axis',(0.,0.,-1.));
#8065=DIRECTION('ref_axis',(-1.,0.,0.));
#8066=DIRECTION('',(1.,0.,0.));
#8067=DIRECTION('',(0.,1.,0.));
#8068=DIRECTION('',(-1.,0.,0.));
#8069=DIRECTION('',(0.,1.,0.));
#8070=DIRECTION('',(1.,0.,0.));
#8071=DIRECTION('',(0.,1.,0.));
#8072=DIRECTION('',(-1.,0.,0.));
#8073=DIRECTION('',(0.,1.,0.));
#8074=DIRECTION('',(1.,0.,0.));
#8075=DIRECTION('',(0.,1.,0.));
#8076=DIRECTION('',(-1.,0.,0.));
#8077=DIRECTION('',(0.,-1.,0.));
#8078=DIRECTION('center_axis',(0.,1.,0.));
#8079=DIRECTION('ref_axis',(0.,0.,1.));
#8080=DIRECTION('',(1.,0.,0.));
#8081=DIRECTION('',(0.,0.,-1.));
#8082=DIRECTION('',(0.,0.,1.));
#8083=DIRECTION('center_axis',(0.,1.,0.));
#8084=DIRECTION('ref_axis',(1.,0.,0.));
#8085=DIRECTION('',(-1.,0.,0.));
#8086=DIRECTION('',(0.,0.,-1.));
#8087=DIRECTION('',(0.,0.,1.));
#8088=DIRECTION('center_axis',(-1.,0.,0.));
#8089=DIRECTION('ref_axis',(0.,0.,1.));
#8090=DIRECTION('',(0.,0.,1.));
#8091=DIRECTION('',(0.,1.,0.));
#8092=DIRECTION('',(0.,0.,-1.));
#8093=DIRECTION('center_axis',(0.,1.,0.));
#8094=DIRECTION('ref_axis',(0.,0.,1.));
#8095=DIRECTION('',(0.,0.,-1.));
#8096=DIRECTION('',(-1.,0.,0.));
#8097=DIRECTION('center_axis',(0.,0.,-1.));
#8098=DIRECTION('ref_axis',(-1.,0.,0.));
#8099=DIRECTION('',(1.,0.,0.));
#8100=DIRECTION('',(0.,1.,0.));
#8101=DIRECTION('center_axis',(1.,0.,0.));
#8102=DIRECTION('ref_axis',(0.,0.,-1.));
#8103=DIRECTION('',(0.,0.,1.));
#8104=DIRECTION('',(0.,1.,0.));
#8105=DIRECTION('center_axis',(0.,1.,0.));
#8106=DIRECTION('ref_axis',(1.,0.,0.));
#8107=DIRECTION('center_axis',(1.,0.,0.));
#8108=DIRECTION('ref_axis',(0.,1.,0.));
#8109=DIRECTION('',(0.,0.,1.));
#8110=DIRECTION('',(0.,1.,0.));
#8111=DIRECTION('',(0.,0.,1.));
#8112=DIRECTION('center_axis',(0.,-1.,0.));
#8113=DIRECTION('ref_axis',(1.,0.,0.));
#8114=DIRECTION('',(0.,0.,1.));
#8115=DIRECTION('',(1.,0.,0.));
#8116=DIRECTION('center_axis',(0.,1.,0.));
#8117=DIRECTION('ref_axis',(-1.,0.,0.));
#8118=DIRECTION('',(-1.,0.,0.));
#8119=DIRECTION('',(0.,0.,1.));
#8120=DIRECTION('center_axis',(-1.,0.,0.));
#8121=DIRECTION('ref_axis',(0.,-1.,0.));
#8122=DIRECTION('',(0.,-1.,0.));
#8123=DIRECTION('',(0.,1.,0.));
#8124=DIRECTION('center_axis',(0.,0.,1.));
#8125=DIRECTION('ref_axis',(1.,0.,0.));
#8126=DIRECTION('center_axis',(0.,0.,1.));
#8127=DIRECTION('ref_axis',(1.,0.,0.));
#9934=CARTESIAN_POINT('',(0.,0.,0.));
#9935=CARTESIAN_POINT('Origin',(-1.06066017177982,-1.06066017177982,13.2));
#9936=CARTESIAN_POINT('',(-1.22566017177982,-1.06066017177982,13.2));
#9937=CARTESIAN_POINT('Origin',(-1.06066017177982,-1.06066017177982,13.2));
#9938=CARTESIAN_POINT('',(-1.22566017177982,-1.06066017177982,14.));
#9939=CARTESIAN_POINT('',(-1.22566017177982,-1.06066017177982,13.2));
#9940=CARTESIAN_POINT('Origin',(-1.06066017177982,-1.06066017177982,14.));
#9941=CARTESIAN_POINT('Origin',(-1.06066017177982,-1.06066017177982,13.2));
#9942=CARTESIAN_POINT('Origin',(-1.06066017177982,1.06066017177982,13.2));
#9943=CARTESIAN_POINT('',(-1.22566017177982,1.06066017177982,13.2));
#9944=CARTESIAN_POINT('Origin',(-1.06066017177982,1.06066017177982,13.2));
#9945=CARTESIAN_POINT('',(-1.22566017177982,1.06066017177982,14.));
#9946=CARTESIAN_POINT('',(-1.22566017177982,1.06066017177982,13.2));
#9947=CARTESIAN_POINT('Origin',(-1.06066017177982,1.06066017177982,14.));
#9948=CARTESIAN_POINT('Origin',(-1.06066017177982,1.06066017177982,13.2));
#9949=CARTESIAN_POINT('Origin',(1.06066017177982,1.06066017177982,13.2));
#9950=CARTESIAN_POINT('',(0.895660171779821,1.06066017177982,13.2));
#9951=CARTESIAN_POINT('Origin',(1.06066017177982,1.06066017177982,13.2));
#9952=CARTESIAN_POINT('',(0.895660171779821,1.06066017177982,14.));
#9953=CARTESIAN_POINT('',(0.895660171779821,1.06066017177982,13.2));
#9954=CARTESIAN_POINT('Origin',(1.06066017177982,1.06066017177982,14.));
#9955=CARTESIAN_POINT('Origin',(1.06066017177982,1.06066017177982,13.2));
#9956=CARTESIAN_POINT('Origin',(1.06066017177982,-1.06066017177982,13.2));
#9957=CARTESIAN_POINT('',(0.895660171779821,-1.06066017177982,13.2));
#9958=CARTESIAN_POINT('Origin',(1.06066017177982,-1.06066017177982,13.2));
#9959=CARTESIAN_POINT('',(0.895660171779821,-1.06066017177982,14.));
#9960=CARTESIAN_POINT('',(0.895660171779821,-1.06066017177982,13.2));
#9961=CARTESIAN_POINT('Origin',(1.06066017177982,-1.06066017177982,14.));
#9962=CARTESIAN_POINT('Origin',(1.06066017177982,-1.06066017177982,13.2));
#9963=CARTESIAN_POINT('Origin',(0.,0.,10.5));
#9964=CARTESIAN_POINT('',(-1.05,-1.28587913910472E-16,10.5));
#9965=CARTESIAN_POINT('Origin',(0.,0.,10.5));
#9966=CARTESIAN_POINT('',(-1.05,1.28587913910472E-16,14.));
#9967=CARTESIAN_POINT('',(-1.05,-1.28587913910472E-16,10.5));
#9968=CARTESIAN_POINT('Origin',(0.,0.,14.));
#9969=CARTESIAN_POINT('Origin',(0.,0.,10.5));
#9970=CARTESIAN_POINT('',(-0.625,-7.65404249467096E-17,10.5));
#9971=CARTESIAN_POINT('Origin',(0.,0.,10.5));
#9972=CARTESIAN_POINT('Origin',(0.,0.,9.9));
#9973=CARTESIAN_POINT('',(-0.625,-7.65404249467096E-17,10.));
#9974=CARTESIAN_POINT('Origin',(0.,0.,10.));
#9975=CARTESIAN_POINT('',(-0.625,-7.65404249467096E-17,9.9));
#9976=CARTESIAN_POINT('Origin',(3.75,0.,2.4));
#9977=CARTESIAN_POINT('',(3.25,-6.12323399573677E-17,2.4));
#9978=CARTESIAN_POINT('Origin',(3.75,0.,2.4));
#9979=CARTESIAN_POINT('',(3.25,6.12323399573677E-17,14.));
#9980=CARTESIAN_POINT('',(3.25,-6.12323399573677E-17,2.4));
#9981=CARTESIAN_POINT('Origin',(3.75,0.,14.));
#9982=CARTESIAN_POINT('Origin',(3.75,0.,2.4));
#9983=CARTESIAN_POINT('',(3.475,-3.36777869765523E-17,2.4));
#9984=CARTESIAN_POINT('Origin',(3.75,0.,2.4));
#9985=CARTESIAN_POINT('Origin',(3.75,0.,0.9));
#9986=CARTESIAN_POINT('',(3.475,-3.36777869765523E-17,1.));
#9987=CARTESIAN_POINT('Origin',(3.75,0.,1.));
#9988=CARTESIAN_POINT('',(3.475,-3.36777869765523E-17,0.9));
#9989=CARTESIAN_POINT('Origin',(-3.75,0.,2.4));
#9990=CARTESIAN_POINT('',(-4.25,-6.12323399573677E-17,2.4));
#9991=CARTESIAN_POINT('Origin',(-3.75,0.,2.4));
#9992=CARTESIAN_POINT('',(-4.25,6.12323399573677E-17,14.));
#9993=CARTESIAN_POINT('',(-4.25,-6.12323399573677E-17,2.4));
#9994=CARTESIAN_POINT('Origin',(-3.75,0.,14.));
#9995=CARTESIAN_POINT('Origin',(-3.75,0.,2.4));
#9996=CARTESIAN_POINT('',(-4.025,-3.36777869765522E-17,2.4));
#9997=CARTESIAN_POINT('Origin',(-3.75,0.,2.4));
#9998=CARTESIAN_POINT('Origin',(-3.75,0.,0.9));
#9999=CARTESIAN_POINT('',(-4.025,-3.36777869765522E-17,1.));
#10000=CARTESIAN_POINT('Origin',(-3.75,0.,1.));
#10001=CARTESIAN_POINT('',(-4.025,-3.36777869765522E-17,0.9));
#10002=CARTESIAN_POINT('Origin',(4.5,-2.,10.));
#10003=CARTESIAN_POINT('',(-4.5,1.,10.));
#10004=CARTESIAN_POINT('',(-3.,1.,10.));
#10005=CARTESIAN_POINT('',(0.75,1.,10.));
#10006=CARTESIAN_POINT('',(-4.5,2.,10.));
#10007=CARTESIAN_POINT('',(-4.5,-2.,10.));
#10008=CARTESIAN_POINT('',(4.5,2.,10.));
#10009=CARTESIAN_POINT('',(-4.5,2.,10.));
#10010=CARTESIAN_POINT('',(4.5,1.,10.));
#10011=CARTESIAN_POINT('',(4.5,-2.,10.));
#10012=CARTESIAN_POINT('',(3.,1.,10.));
#10013=CARTESIAN_POINT('',(4.125,1.,10.));
#10014=CARTESIAN_POINT('',(3.,-1.,10.));
#10015=CARTESIAN_POINT('',(3.,-1.5,10.));
#10016=CARTESIAN_POINT('',(4.5,-1.,10.));
#10017=CARTESIAN_POINT('',(4.125,-1.,10.));
#10018=CARTESIAN_POINT('',(4.5,-2.,10.));
#10019=CARTESIAN_POINT('',(4.5,-2.,10.));
#10020=CARTESIAN_POINT('',(-4.5,-2.,10.));
#10021=CARTESIAN_POINT('',(-4.5,-2.,10.));
#10022=CARTESIAN_POINT('',(-4.5,-1.,10.));
#10023=CARTESIAN_POINT('',(-4.5,-2.,10.));
#10024=CARTESIAN_POINT('',(-3.,-1.,10.));
#10025=CARTESIAN_POINT('',(0.,-1.,10.));
#10026=CARTESIAN_POINT('',(-3.,-1.5,10.));
#10027=CARTESIAN_POINT('Origin',(0.,2.,12.));
#10028=CARTESIAN_POINT('',(-4.5,2.,14.));
#10029=CARTESIAN_POINT('',(4.5,2.,14.));
#10030=CARTESIAN_POINT('',(4.5,2.,14.));
#10031=CARTESIAN_POINT('',(4.5,2.,10.));
#10032=CARTESIAN_POINT('',(-4.5,2.,14.));
#10033=CARTESIAN_POINT('Origin',(0.,-2.,12.));
#10034=CARTESIAN_POINT('',(4.5,-2.,14.));
#10035=CARTESIAN_POINT('',(-4.5,-2.,14.));
#10036=CARTESIAN_POINT('',(4.5,-2.,14.));
#10037=CARTESIAN_POINT('',(-4.5,-2.,14.));
#10038=CARTESIAN_POINT('',(4.5,-2.,10.));
#10039=CARTESIAN_POINT('Origin',(3.,-1.,1.));
#10040=CARTESIAN_POINT('',(3.,1.,1.));
#10041=CARTESIAN_POINT('',(3.,1.,14.));
#10042=CARTESIAN_POINT('',(3.,-1.,1.));
#10043=CARTESIAN_POINT('',(3.,-1.,1.));
#10044=CARTESIAN_POINT('',(3.,-1.,14.));
#10045=CARTESIAN_POINT('Origin',(3.75,1.,7.5));
#10046=CARTESIAN_POINT('',(4.5,1.,1.));
#10047=CARTESIAN_POINT('',(4.5,1.,1.));
#10048=CARTESIAN_POINT('',(3.,1.,1.));
#10049=CARTESIAN_POINT('Origin',(4.5,-1.,1.));
#10050=CARTESIAN_POINT('',(4.5,-1.,1.));
#10051=CARTESIAN_POINT('',(3.,-1.,1.));
#10052=CARTESIAN_POINT('',(4.5,-1.,1.));
#10053=CARTESIAN_POINT('Origin',(4.5,-1.,14.));
#10054=CARTESIAN_POINT('',(4.5,-1.,1.));
#10055=CARTESIAN_POINT('',(4.5,-1.,14.));
#10056=CARTESIAN_POINT('Origin',(3.75,-1.,7.5));
#10057=CARTESIAN_POINT('Origin',(-3.,-1.,1.));
#10058=CARTESIAN_POINT('',(-3.,-1.,1.));
#10059=CARTESIAN_POINT('',(-3.,-1.,1.));
#10060=CARTESIAN_POINT('',(-3.,1.,1.));
#10061=CARTESIAN_POINT('',(-3.,-1.,1.));
#10062=CARTESIAN_POINT('',(-3.,1.,1.));
#10063=CARTESIAN_POINT('Origin',(-4.5,-1.,1.));
#10064=CARTESIAN_POINT('',(-4.5,-1.,1.));
#10065=CARTESIAN_POINT('',(-4.5,-1.,1.));
#10066=CARTESIAN_POINT('',(-4.5,-1.,1.));
#10067=CARTESIAN_POINT('Origin',(-3.,1.,1.));
#10068=CARTESIAN_POINT('',(-4.5,1.,1.));
#10069=CARTESIAN_POINT('',(-3.,1.,1.));
#10070=CARTESIAN_POINT('',(-4.5,1.,1.));
#10071=CARTESIAN_POINT('Origin',(-4.5,1.,1.));
#10072=CARTESIAN_POINT('',(-4.5,1.,1.));
#10073=CARTESIAN_POINT('',(-4.5,-2.,14.));
#10074=CARTESIAN_POINT('Origin',(-3.75,0.,14.));
#10075=CARTESIAN_POINT('Origin',(-3.75,0.,1.));
#12822=UNCERTAINTY_MEASURE_WITH_UNIT(LENGTH_MEASURE(0.001),#12897,
'DISTANCE_ACCURACY_VALUE',
'Maximum model space distance between geometric entities at asserted c
onnectivities');
#12853=UNCERTAINTY_MEASURE_WITH_UNIT(LENGTH_MEASURE(0.001),#12897,
'DISTANCE_ACCURACY_VALUE',
'Maximum model space distance between geometric entities at asserted c
onnectivities');
#12865=(
GEOMETRIC_REPRESENTATION_CONTEXT(3)
GLOBAL_UNCERTAINTY_ASSIGNED_CONTEXT((#12822))
GLOBAL_UNIT_ASSIGNED_CONTEXT((#12897,#12899,#12900))
REPRESENTATION_CONTEXT('','3D')
);
#12896=(
GEOMETRIC_REPRESENTATION_CONTEXT(3)
GLOBAL_UNCERTAINTY_ASSIGNED_CONTEXT((#12853))
GLOBAL_UNIT_ASSIGNED_CONTEXT((#12897,#12899,#12900))
REPRESENTATION_CONTEXT('','3D')
);
#12897=(
LENGTH_UNIT()
NAMED_UNIT(*)
SI_UNIT(.CENTI.,.METRE.)
);
#12899=(
NAMED_UNIT(*)
PLANE_ANGLE_UNIT()
SI_UNIT($,.RADIAN.)
);
#12900=(
NAMED_UNIT(*)
SI_UNIT($,.STERADIAN.)
SOLID_ANGLE_UNIT()
);
#12912=SHAPE_DEFINITION_REPRESENTATION(#12954,#13065);
#12954=PRODUCT_DEFINITION_SHAPE('',$,#13108);
#13065=SHAPE_REPRESENTATION('',(#6832),#12865);
#13096=PRODUCT_DEFINITION_CONTEXT('part definition',#13224,'design');
#13108=PRODUCT_DEFINITION('Valve guide bridge','Valve guide bridge',#13150,
#13096);
#13150=PRODUCT_DEFINITION_FORMATION('',$,#13237);
#13224=APPLICATION_CONTEXT(
'Core Data for Automotive Mechanical Design Process');
#13225=PRODUCT_CONTEXT('part definition',#13224,'mechanical');
#13237=PRODUCT('Valve guide bridge','Valve guide bridge',
'Valve guide bridge',(#13225));
#13317=COLOUR_RGB('Sky Blue',0.24,0.69,0.87);
#13318=FILL_AREA_STYLE_COLOUR('',#13317);
#13319=FILL_AREA_STYLE('',(#13318));
#13320=SURFACE_STYLE_FILL_AREA(#13319);
#13321=SURFACE_SIDE_STYLE('',(#13320));
#13322=SURFACE_STYLE_USAGE(.BOTH.,#13321);
#13323=PRESENTATION_STYLE_ASSIGNMENT((#13322));
ENDSEC;
END-ISO-10303-21;
